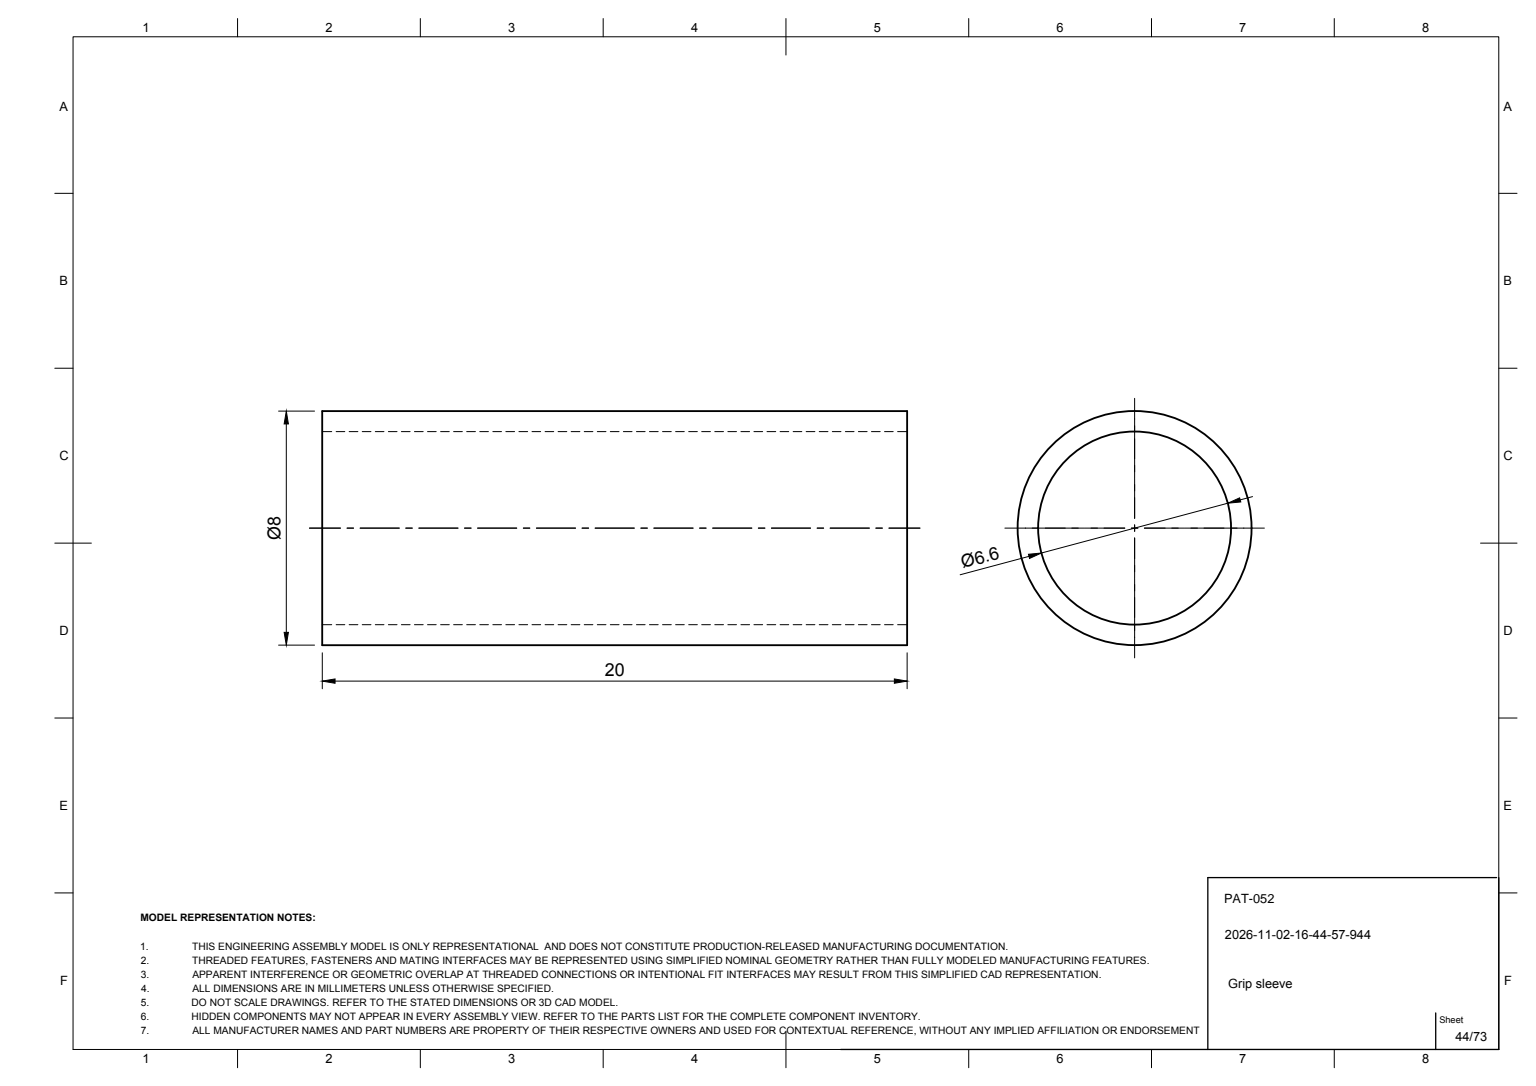
ISO-10303-21;
HEADER;
/* Generated by software containing ST-Developer
 * from STEP Tools, Inc. (www.steptools.com) 
 */

FILE_DESCRIPTION(
/* description */ ('Hand-crank gear train demonstrator'),
/* implementation_level */ '2;1');

FILE_NAME(
/* name */ 'Grip sleeve.step',
/* time_stamp */ '2026-10-28T03:22:13-07:00',
/* author */ (''),
/* organization */ (''),
/* preprocessor_version */ 'ST-DEVELOPER v20.2',
/* originating_system */ 'Autodesk Translation Framework v15.17.0.0',
/* authorisation */ '');

FILE_SCHEMA (('AUTOMOTIVE_DESIGN { 1 0 10303 214 3 1 1 }'));
ENDSEC;

DATA;
#10=MECHANICAL_DESIGN_GEOMETRIC_PRESENTATION_REPRESENTATION('',(#1240),#62758);
#1097=SHAPE_REPRESENTATION_RELATIONSHIP('SRR','None',#63072,#1161);
#1161=ADVANCED_BREP_SHAPE_REPRESENTATION('',(#1316),#62726);
#1240=STYLED_ITEM('',(#63469),#1316);
#1316=MANIFOLD_SOLID_BREP('Body1',#16423);
#1566=FACE_BOUND('',#3769,.T.);
#1567=FACE_BOUND('',#3771,.T.);
#1921=PLANE('',#18096);
#1922=PLANE('',#18097);
#2606=FACE_OUTER_BOUND('',#3766,.T.);
#2607=FACE_OUTER_BOUND('',#3767,.T.);
#2608=FACE_OUTER_BOUND('',#3768,.T.);
#2609=FACE_OUTER_BOUND('',#3770,.T.);
#3766=EDGE_LOOP('',(#12933,#12934,#12935,#12936));
#3767=EDGE_LOOP('',(#12937,#12938,#12939,#12940));
#3768=EDGE_LOOP('',(#12941));
#3769=EDGE_LOOP('',(#12942));
#3770=EDGE_LOOP('',(#12943));
#3771=EDGE_LOOP('',(#12944));
#4902=LINE('',#26295,#6034);
#4903=LINE('',#26301,#6035);
#6034=VECTOR('',#21315,0.33);
#6035=VECTOR('',#21322,0.4);
#6947=CIRCLE('',#18091,0.33);
#6948=CIRCLE('',#18092,0.33);
#6949=CIRCLE('',#18094,0.4);
#6950=CIRCLE('',#18095,0.4);
#7926=VERTEX_POINT('',#26292);
#7927=VERTEX_POINT('',#26294);
#7928=VERTEX_POINT('',#26298);
#7929=VERTEX_POINT('',#26300);
#9718=EDGE_CURVE('',#7926,#7926,#6947,.T.);
#9719=EDGE_CURVE('',#7926,#7927,#4902,.T.);
#9720=EDGE_CURVE('',#7927,#7927,#6948,.T.);
#9721=EDGE_CURVE('',#7928,#7928,#6949,.T.);
#9722=EDGE_CURVE('',#7928,#7929,#4903,.T.);
#9723=EDGE_CURVE('',#7929,#7929,#6950,.T.);
#12933=ORIENTED_EDGE('',*,*,#9718,.F.);
#12934=ORIENTED_EDGE('',*,*,#9719,.T.);
#12935=ORIENTED_EDGE('',*,*,#9720,.T.);
#12936=ORIENTED_EDGE('',*,*,#9719,.F.);
#12937=ORIENTED_EDGE('',*,*,#9721,.F.);
#12938=ORIENTED_EDGE('',*,*,#9722,.T.);
#12939=ORIENTED_EDGE('',*,*,#9723,.T.);
#12940=ORIENTED_EDGE('',*,*,#9722,.F.);
#12941=ORIENTED_EDGE('',*,*,#9721,.T.);
#12942=ORIENTED_EDGE('',*,*,#9718,.T.);
#12943=ORIENTED_EDGE('',*,*,#9723,.F.);
#12944=ORIENTED_EDGE('',*,*,#9720,.F.);
#15311=CYLINDRICAL_SURFACE('',#18090,0.33);
#15312=CYLINDRICAL_SURFACE('',#18093,0.4);
#15916=ADVANCED_FACE('',(#2606),#15311,.F.);
#15917=ADVANCED_FACE('',(#2607),#15312,.T.);
#15918=ADVANCED_FACE('',(#2608,#1566),#1921,.T.);
#15919=ADVANCED_FACE('',(#2609,#1567),#1922,.F.);
#16423=CLOSED_SHELL('',(#15916,#15917,#15918,#15919));
#18089=AXIS2_PLACEMENT_3D('',#26290,#21309,#21310);
#18090=AXIS2_PLACEMENT_3D('',#26291,#21311,#21312);
#18091=AXIS2_PLACEMENT_3D('',#26293,#21313,#21314);
#18092=AXIS2_PLACEMENT_3D('',#26296,#21316,#21317);
#18093=AXIS2_PLACEMENT_3D('',#26297,#21318,#21319);
#18094=AXIS2_PLACEMENT_3D('',#26299,#21320,#21321);
#18095=AXIS2_PLACEMENT_3D('',#26302,#21323,#21324);
#18096=AXIS2_PLACEMENT_3D('',#26303,#21325,#21326);
#18097=AXIS2_PLACEMENT_3D('',#26304,#21327,#21328);
#21309=DIRECTION('axis',(0.,0.,1.));
#21310=DIRECTION('refdir',(1.,0.,0.));
#21311=DIRECTION('center_axis',(0.,1.,0.));
#21312=DIRECTION('ref_axis',(1.,0.,0.));
#21313=DIRECTION('center_axis',(0.,-1.,0.));
#21314=DIRECTION('ref_axis',(1.,0.,0.));
#21315=DIRECTION('',(0.,-1.,0.));
#21316=DIRECTION('center_axis',(0.,-1.,0.));
#21317=DIRECTION('ref_axis',(1.,0.,0.));
#21318=DIRECTION('center_axis',(0.,1.,0.));
#21319=DIRECTION('ref_axis',(1.,0.,0.));
#21320=DIRECTION('center_axis',(0.,1.,0.));
#21321=DIRECTION('ref_axis',(1.,0.,0.));
#21322=DIRECTION('',(0.,-1.,0.));
#21323=DIRECTION('center_axis',(0.,1.,0.));
#21324=DIRECTION('ref_axis',(1.,0.,0.));
#21325=DIRECTION('center_axis',(0.,1.,0.));
#21326=DIRECTION('ref_axis',(1.,0.,0.));
#21327=DIRECTION('center_axis',(0.,1.,0.));
#21328=DIRECTION('ref_axis',(1.,0.,0.));
#26290=CARTESIAN_POINT('',(0.,0.,0.));
#26291=CARTESIAN_POINT('Origin',(0.,4.8,13.));
#26292=CARTESIAN_POINT('',(-0.33,6.8,13.));
#26293=CARTESIAN_POINT('Origin',(0.,6.8,13.));
#26294=CARTESIAN_POINT('',(-0.33,4.8,13.));
#26295=CARTESIAN_POINT('',(-0.33,4.8,13.));
#26296=CARTESIAN_POINT('Origin',(0.,4.8,13.));
#26297=CARTESIAN_POINT('Origin',(0.,4.8,13.));
#26298=CARTESIAN_POINT('',(-0.4,6.8,13.));
#26299=CARTESIAN_POINT('Origin',(0.,6.8,13.));
#26300=CARTESIAN_POINT('',(-0.4,4.8,13.));
#26301=CARTESIAN_POINT('',(-0.4,4.8,13.));
#26302=CARTESIAN_POINT('Origin',(0.,4.8,13.));
#26303=CARTESIAN_POINT('Origin',(0.,6.8,13.));
#26304=CARTESIAN_POINT('Origin',(0.,4.8,13.));
#62652=UNCERTAINTY_MEASURE_WITH_UNIT(LENGTH_MEASURE(0.001),#62759,
'DISTANCE_ACCURACY_VALUE',
'Maximum model space distance between geometric entities at asserted c
onnectivities');
#62684=UNCERTAINTY_MEASURE_WITH_UNIT(LENGTH_MEASURE(0.001),#62759,
'DISTANCE_ACCURACY_VALUE',
'Maximum model space distance between geometric entities at asserted c
onnectivities');
#62726=(
GEOMETRIC_REPRESENTATION_CONTEXT(3)
GLOBAL_UNCERTAINTY_ASSIGNED_CONTEXT((#62652))
GLOBAL_UNIT_ASSIGNED_CONTEXT((#62759,#62761,#62762))
REPRESENTATION_CONTEXT('','3D')
);
#62758=(
GEOMETRIC_REPRESENTATION_CONTEXT(3)
GLOBAL_UNCERTAINTY_ASSIGNED_CONTEXT((#62684))
GLOBAL_UNIT_ASSIGNED_CONTEXT((#62759,#62761,#62762))
REPRESENTATION_CONTEXT('','3D')
);
#62759=(
LENGTH_UNIT()
NAMED_UNIT(*)
SI_UNIT(.CENTI.,.METRE.)
);
#62761=(
NAMED_UNIT(*)
PLANE_ANGLE_UNIT()
SI_UNIT($,.RADIAN.)
);
#62762=(
NAMED_UNIT(*)
SI_UNIT($,.STERADIAN.)
SOLID_ANGLE_UNIT()
);
#62804=SHAPE_DEFINITION_REPRESENTATION(#62887,#63072);
#62887=PRODUCT_DEFINITION_SHAPE('',$,#63146);
#63072=SHAPE_REPRESENTATION('',(#18089),#62726);
#63104=PRODUCT_DEFINITION_CONTEXT('part definition',#63325,'design');
#63146=PRODUCT_DEFINITION('Grip sleeve','Grip sleeve',#63219,#63104);
#63219=PRODUCT_DEFINITION_FORMATION('',$,#63368);
#63325=APPLICATION_CONTEXT(
'Core Data for Automotive Mechanical Design Process');
#63326=PRODUCT_CONTEXT('part definition',#63325,'mechanical');
#63368=PRODUCT('Grip sleeve','Grip sleeve','Grip sleeve',(#63326));
#63463=COLOUR_RGB('Black',0.12,0.14,0.17);
#63464=FILL_AREA_STYLE_COLOUR('',#63463);
#63465=FILL_AREA_STYLE('',(#63464));
#63466=SURFACE_STYLE_FILL_AREA(#63465);
#63467=SURFACE_SIDE_STYLE('',(#63466));
#63468=SURFACE_STYLE_USAGE(.BOTH.,#63467);
#63469=PRESENTATION_STYLE_ASSIGNMENT((#63468));
ENDSEC;
END-ISO-10303-21;
